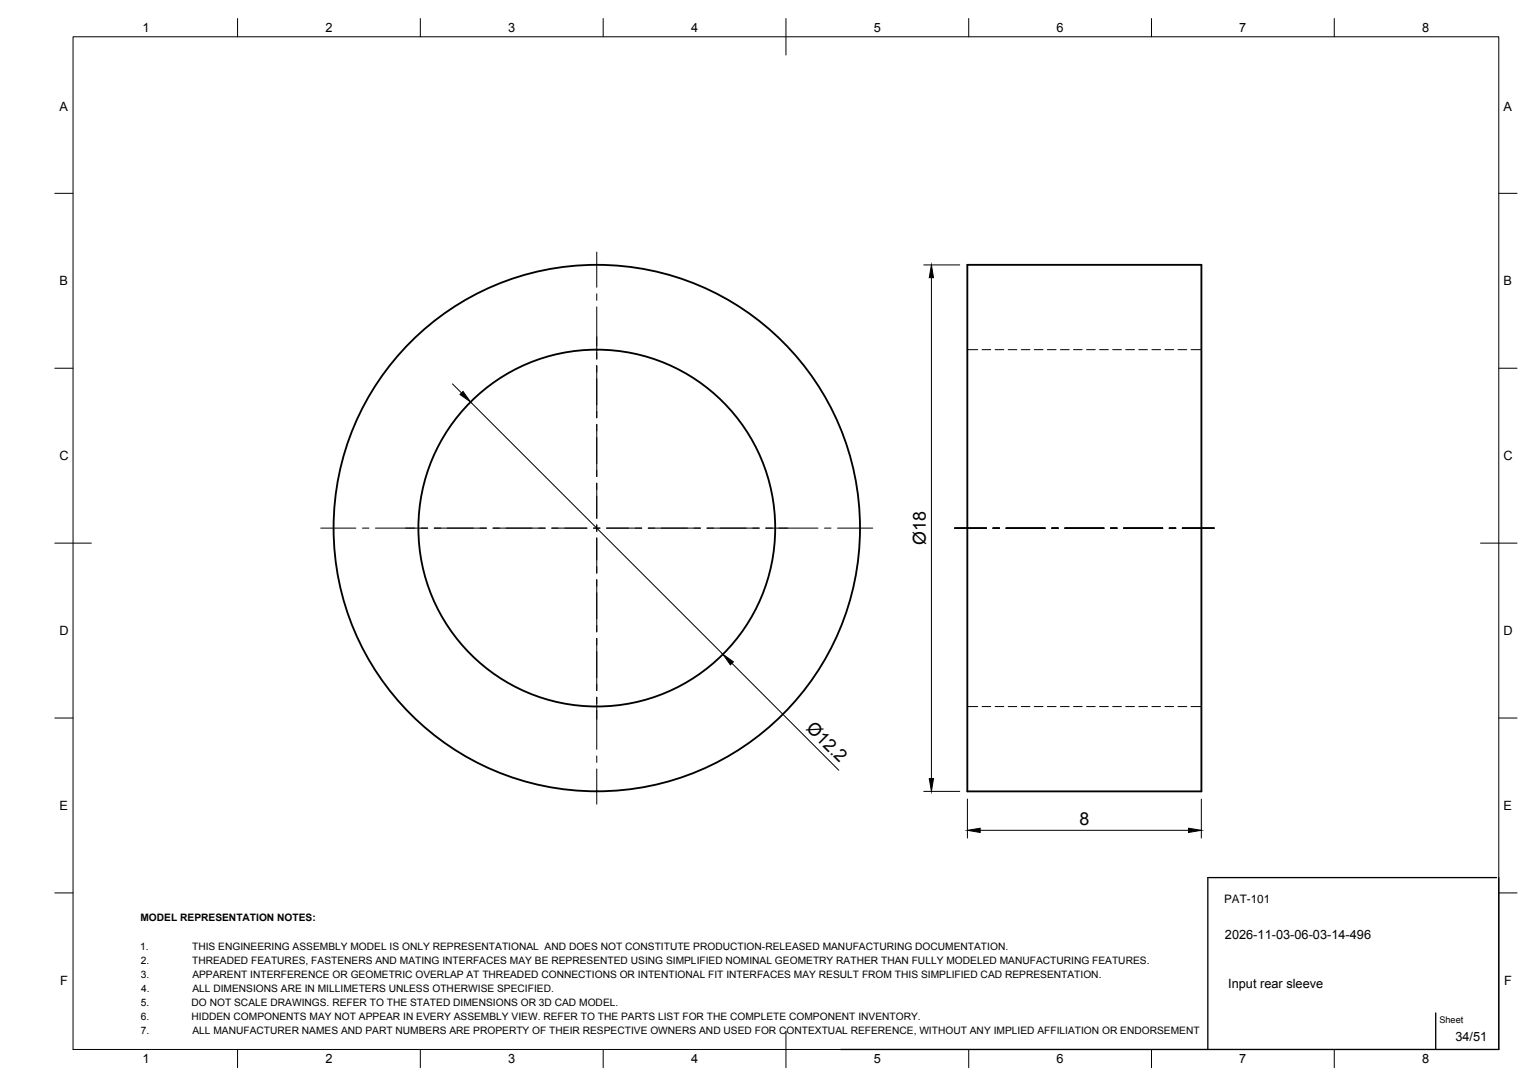
ISO-10303-21;
HEADER;
/* Generated by software containing ST-Developer
 * from STEP Tools, Inc. (www.steptools.com) 
 */

FILE_DESCRIPTION(
/* description */ ('Spur gear reduction stage 2-1 on bearing plates'),
/* implementation_level */ '2;1');

FILE_NAME(
/* name */ 'Input rear sleeve.step',
/* time_stamp */ '2026-10-28T03:22:07-07:00',
/* author */ (''),
/* organization */ (''),
/* preprocessor_version */ 'ST-DEVELOPER v20.2',
/* originating_system */ 'Autodesk Translation Framework v15.17.0.0',
/* authorisation */ '');

FILE_SCHEMA (('AUTOMOTIVE_DESIGN { 1 0 10303 214 3 1 1 }'));
ENDSEC;

DATA;
#10=MECHANICAL_DESIGN_GEOMETRIC_PRESENTATION_REPRESENTATION('',(#988),#53909);
#887=SHAPE_REPRESENTATION_RELATIONSHIP('SRR','None',#54117,#930);
#930=ADVANCED_BREP_SHAPE_REPRESENTATION('',(#1043),#53891);
#988=STYLED_ITEM('',(#54390),#1043);
#1043=MANIFOLD_SOLID_BREP('Body1',#11315);
#1200=FACE_BOUND('',#2586,.T.);
#1201=FACE_BOUND('',#2588,.T.);
#1367=PLANE('',#12510);
#1368=PLANE('',#12511);
#1795=FACE_OUTER_BOUND('',#2583,.T.);
#1796=FACE_OUTER_BOUND('',#2584,.T.);
#1797=FACE_OUTER_BOUND('',#2585,.T.);
#1798=FACE_OUTER_BOUND('',#2587,.T.);
#2583=EDGE_LOOP('',(#8524,#8525,#8526,#8527));
#2584=EDGE_LOOP('',(#8528,#8529,#8530,#8531));
#2585=EDGE_LOOP('',(#8532));
#2586=EDGE_LOOP('',(#8533));
#2587=EDGE_LOOP('',(#8534));
#2588=EDGE_LOOP('',(#8535));
#3206=LINE('',#17974,#3847);
#3207=LINE('',#17980,#3848);
#3847=VECTOR('',#14611,0.61);
#3848=VECTOR('',#14618,0.9);
#4584=CIRCLE('',#12505,0.61);
#4585=CIRCLE('',#12506,0.61);
#4586=CIRCLE('',#12508,0.9);
#4587=CIRCLE('',#12509,0.9);
#5188=VERTEX_POINT('',#17971);
#5189=VERTEX_POINT('',#17973);
#5190=VERTEX_POINT('',#17977);
#5191=VERTEX_POINT('',#17979);
#6404=EDGE_CURVE('',#5188,#5188,#4584,.T.);
#6405=EDGE_CURVE('',#5188,#5189,#3206,.T.);
#6406=EDGE_CURVE('',#5189,#5189,#4585,.T.);
#6407=EDGE_CURVE('',#5190,#5190,#4586,.T.);
#6408=EDGE_CURVE('',#5190,#5191,#3207,.T.);
#6409=EDGE_CURVE('',#5191,#5191,#4587,.T.);
#8524=ORIENTED_EDGE('',*,*,#6404,.F.);
#8525=ORIENTED_EDGE('',*,*,#6405,.T.);
#8526=ORIENTED_EDGE('',*,*,#6406,.T.);
#8527=ORIENTED_EDGE('',*,*,#6405,.F.);
#8528=ORIENTED_EDGE('',*,*,#6407,.F.);
#8529=ORIENTED_EDGE('',*,*,#6408,.T.);
#8530=ORIENTED_EDGE('',*,*,#6409,.T.);
#8531=ORIENTED_EDGE('',*,*,#6408,.F.);
#8532=ORIENTED_EDGE('',*,*,#6407,.T.);
#8533=ORIENTED_EDGE('',*,*,#6404,.T.);
#8534=ORIENTED_EDGE('',*,*,#6409,.F.);
#8535=ORIENTED_EDGE('',*,*,#6406,.F.);
#10529=CYLINDRICAL_SURFACE('',#12504,0.61);
#10530=CYLINDRICAL_SURFACE('',#12507,0.9);
#10915=ADVANCED_FACE('',(#1795),#10529,.F.);
#10916=ADVANCED_FACE('',(#1796),#10530,.T.);
#10917=ADVANCED_FACE('',(#1797,#1200),#1367,.T.);
#10918=ADVANCED_FACE('',(#1798,#1201),#1368,.F.);
#11315=CLOSED_SHELL('',(#10915,#10916,#10917,#10918));
#12503=AXIS2_PLACEMENT_3D('',#17969,#14605,#14606);
#12504=AXIS2_PLACEMENT_3D('',#17970,#14607,#14608);
#12505=AXIS2_PLACEMENT_3D('',#17972,#14609,#14610);
#12506=AXIS2_PLACEMENT_3D('',#17975,#14612,#14613);
#12507=AXIS2_PLACEMENT_3D('',#17976,#14614,#14615);
#12508=AXIS2_PLACEMENT_3D('',#17978,#14616,#14617);
#12509=AXIS2_PLACEMENT_3D('',#17981,#14619,#14620);
#12510=AXIS2_PLACEMENT_3D('',#17982,#14621,#14622);
#12511=AXIS2_PLACEMENT_3D('',#17983,#14623,#14624);
#14605=DIRECTION('axis',(0.,0.,1.));
#14606=DIRECTION('refdir',(1.,0.,0.));
#14607=DIRECTION('center_axis',(0.,1.,0.));
#14608=DIRECTION('ref_axis',(1.,0.,0.));
#14609=DIRECTION('center_axis',(0.,-1.,0.));
#14610=DIRECTION('ref_axis',(1.,0.,0.));
#14611=DIRECTION('',(0.,-1.,0.));
#14612=DIRECTION('center_axis',(0.,-1.,0.));
#14613=DIRECTION('ref_axis',(1.,0.,0.));
#14614=DIRECTION('center_axis',(0.,1.,0.));
#14615=DIRECTION('ref_axis',(1.,0.,0.));
#14616=DIRECTION('center_axis',(0.,1.,0.));
#14617=DIRECTION('ref_axis',(1.,0.,0.));
#14618=DIRECTION('',(0.,-1.,0.));
#14619=DIRECTION('center_axis',(0.,1.,0.));
#14620=DIRECTION('ref_axis',(1.,0.,0.));
#14621=DIRECTION('center_axis',(0.,1.,0.));
#14622=DIRECTION('ref_axis',(1.,0.,0.));
#14623=DIRECTION('center_axis',(0.,1.,0.));
#14624=DIRECTION('ref_axis',(1.,0.,0.));
#17969=CARTESIAN_POINT('',(0.,0.,0.));
#17970=CARTESIAN_POINT('Origin',(0.,2.2,0.));
#17971=CARTESIAN_POINT('',(-0.61,3.,7.47034547479885E-17));
#17972=CARTESIAN_POINT('Origin',(0.,3.,0.));
#17973=CARTESIAN_POINT('',(-0.61,2.2,7.47034547479885E-17));
#17974=CARTESIAN_POINT('',(-0.61,2.2,7.47034547479885E-17));
#17975=CARTESIAN_POINT('Origin',(0.,2.2,0.));
#17976=CARTESIAN_POINT('Origin',(0.,2.2,0.));
#17977=CARTESIAN_POINT('',(-0.9,3.,1.10218211923262E-16));
#17978=CARTESIAN_POINT('Origin',(0.,3.,0.));
#17979=CARTESIAN_POINT('',(-0.9,2.2,1.10218211923262E-16));
#17980=CARTESIAN_POINT('',(-0.9,2.2,1.10218211923262E-16));
#17981=CARTESIAN_POINT('Origin',(0.,2.2,0.));
#17982=CARTESIAN_POINT('Origin',(0.,3.,0.));
#17983=CARTESIAN_POINT('Origin',(0.,2.2,0.));
#53841=UNCERTAINTY_MEASURE_WITH_UNIT(LENGTH_MEASURE(0.001),#53910,
'DISTANCE_ACCURACY_VALUE',
'Maximum model space distance between geometric entities at asserted c
onnectivities');
#53859=UNCERTAINTY_MEASURE_WITH_UNIT(LENGTH_MEASURE(0.001),#53910,
'DISTANCE_ACCURACY_VALUE',
'Maximum model space distance between geometric entities at asserted c
onnectivities');
#53891=(
GEOMETRIC_REPRESENTATION_CONTEXT(3)
GLOBAL_UNCERTAINTY_ASSIGNED_CONTEXT((#53841))
GLOBAL_UNIT_ASSIGNED_CONTEXT((#53910,#53912,#53913))
REPRESENTATION_CONTEXT('','3D')
);
#53909=(
GEOMETRIC_REPRESENTATION_CONTEXT(3)
GLOBAL_UNCERTAINTY_ASSIGNED_CONTEXT((#53859))
GLOBAL_UNIT_ASSIGNED_CONTEXT((#53910,#53912,#53913))
REPRESENTATION_CONTEXT('','3D')
);
#53910=(
LENGTH_UNIT()
NAMED_UNIT(*)
SI_UNIT(.CENTI.,.METRE.)
);
#53912=(
NAMED_UNIT(*)
PLANE_ANGLE_UNIT()
SI_UNIT($,.RADIAN.)
);
#53913=(
NAMED_UNIT(*)
SI_UNIT($,.STERADIAN.)
SOLID_ANGLE_UNIT()
);
#53945=SHAPE_DEFINITION_REPRESENTATION(#54043,#54117);
#54043=PRODUCT_DEFINITION_SHAPE('',$,#54167);
#54117=SHAPE_REPRESENTATION('',(#12503),#53891);
#54135=PRODUCT_DEFINITION_CONTEXT('part definition',#54284,'design');
#54167=PRODUCT_DEFINITION('Input rear sleeve','Input rear sleeve',#54216,
#54135);
#54216=PRODUCT_DEFINITION_FORMATION('',$,#54317);
#54284=APPLICATION_CONTEXT(
'Core Data for Automotive Mechanical Design Process');
#54285=PRODUCT_CONTEXT('part definition',#54284,'mechanical');
#54317=PRODUCT('Input rear sleeve','Input rear sleeve',
'Input rear sleeve',(#54285));
#54384=COLOUR_RGB('Sky Blue',0.24,0.69,0.87);
#54385=FILL_AREA_STYLE_COLOUR('',#54384);
#54386=FILL_AREA_STYLE('',(#54385));
#54387=SURFACE_STYLE_FILL_AREA(#54386);
#54388=SURFACE_SIDE_STYLE('',(#54387));
#54389=SURFACE_STYLE_USAGE(.BOTH.,#54388);
#54390=PRESENTATION_STYLE_ASSIGNMENT((#54389));
ENDSEC;
END-ISO-10303-21;
